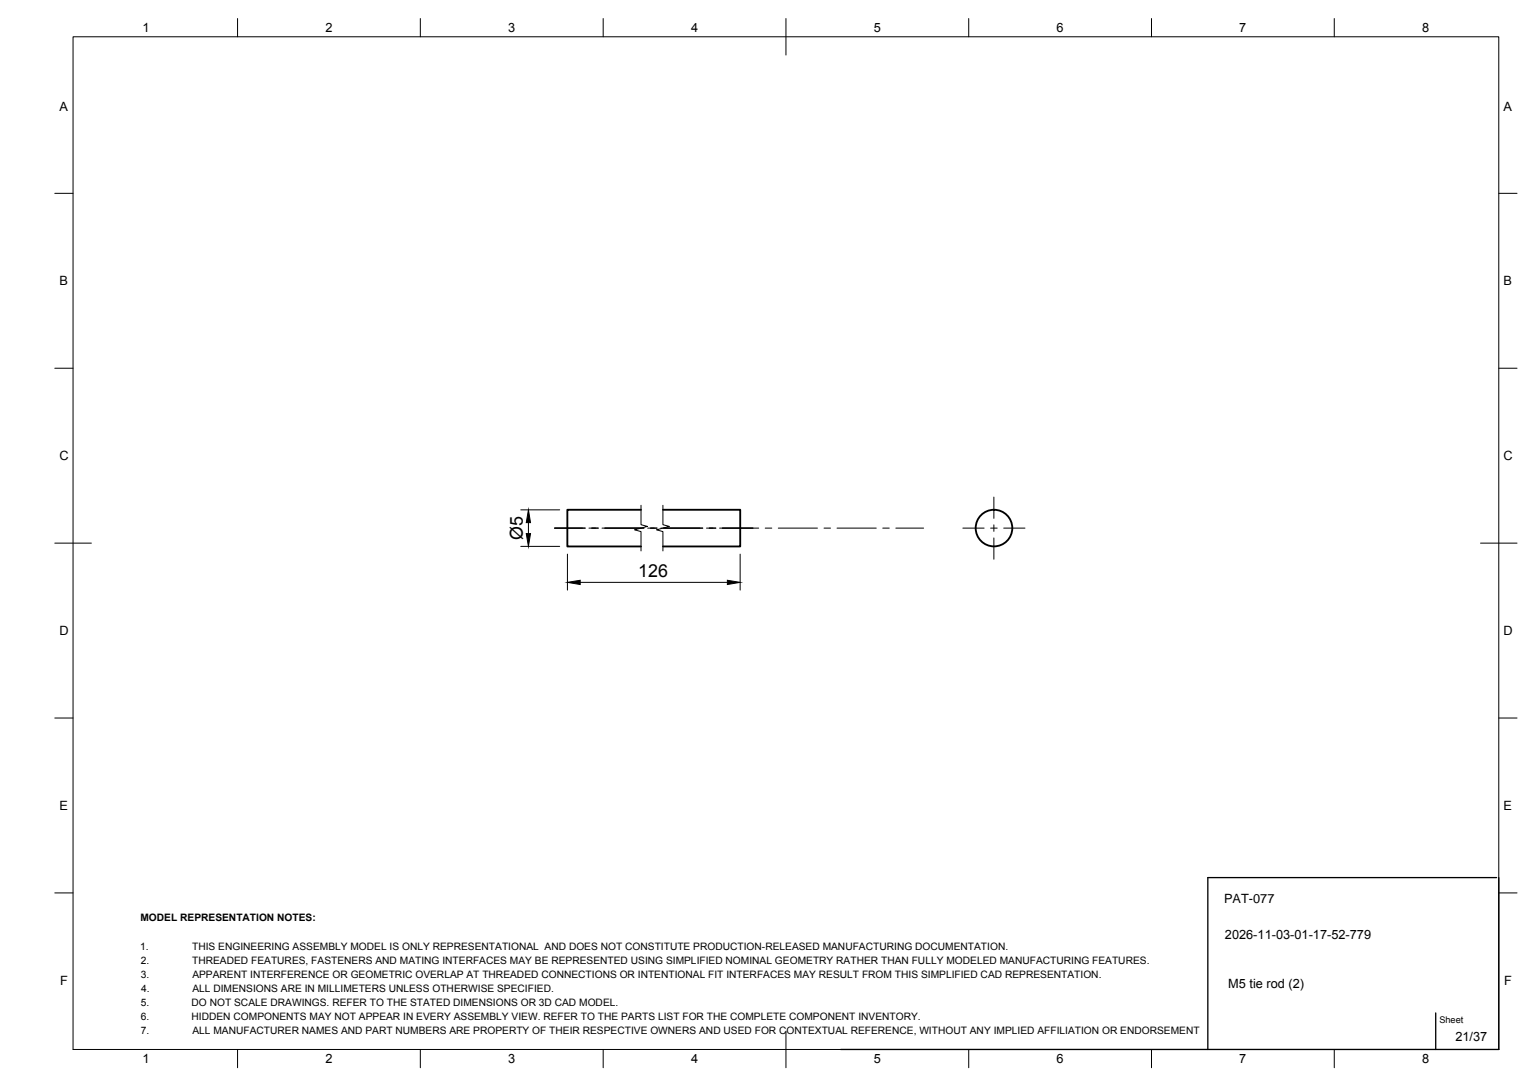
ISO-10303-21;
HEADER;
/* Generated by software containing ST-Developer
 * from STEP Tools, Inc. (www.steptools.com) 
 */

FILE_DESCRIPTION(
/* description */ ('Pallet stop with pneumatic fitting'),
/* implementation_level */ '2;1');

FILE_NAME(
/* name */ 'M5 tie rod (2).step',
/* time_stamp */ '2026-10-27T10:51:41-07:00',
/* author */ (''),
/* organization */ (''),
/* preprocessor_version */ 'ST-DEVELOPER v20.2',
/* originating_system */ 'Autodesk Translation Framework v15.17.0.0',
/* authorisation */ '');

FILE_SCHEMA (('AUTOMOTIVE_DESIGN { 1 0 10303 214 3 1 1 }'));
ENDSEC;

DATA;
#10=MECHANICAL_DESIGN_GEOMETRIC_PRESENTATION_REPRESENTATION('',(#373),#10265);
#309=SHAPE_REPRESENTATION_RELATIONSHIP('SRR','None',#10422,#341);
#341=ADVANCED_BREP_SHAPE_REPRESENTATION('',(#405),#10246);
#373=STYLED_ITEM('',(#10655),#405);
#405=MANIFOLD_SOLID_BREP('Body1',#5061);
#628=PLANE('',#5743);
#629=PLANE('',#5744);
#888=FACE_OUTER_BOUND('',#1287,.T.);
#889=FACE_OUTER_BOUND('',#1288,.T.);
#890=FACE_OUTER_BOUND('',#1289,.T.);
#1287=EDGE_LOOP('',(#3988,#3989,#3990,#3991));
#1288=EDGE_LOOP('',(#3992));
#1289=EDGE_LOOP('',(#3993));
#1634=LINE('',#9346,#1969);
#1969=VECTOR('',#6853,0.25);
#2298=CIRCLE('',#5741,0.25);
#2299=CIRCLE('',#5742,0.25);
#2598=VERTEX_POINT('',#9343);
#2599=VERTEX_POINT('',#9345);
#3093=EDGE_CURVE('',#2598,#2598,#2298,.T.);
#3094=EDGE_CURVE('',#2598,#2599,#1634,.T.);
#3095=EDGE_CURVE('',#2599,#2599,#2299,.T.);
#3988=ORIENTED_EDGE('',*,*,#3093,.F.);
#3989=ORIENTED_EDGE('',*,*,#3094,.T.);
#3990=ORIENTED_EDGE('',*,*,#3095,.T.);
#3991=ORIENTED_EDGE('',*,*,#3094,.F.);
#3992=ORIENTED_EDGE('',*,*,#3093,.T.);
#3993=ORIENTED_EDGE('',*,*,#3095,.F.);
#4690=CYLINDRICAL_SURFACE('',#5740,0.25);
#4883=ADVANCED_FACE('',(#888),#4690,.T.);
#4884=ADVANCED_FACE('',(#889),#628,.T.);
#4885=ADVANCED_FACE('',(#890),#629,.F.);
#5061=CLOSED_SHELL('',(#4883,#4884,#4885));
#5739=AXIS2_PLACEMENT_3D('',#9341,#6847,#6848);
#5740=AXIS2_PLACEMENT_3D('',#9342,#6849,#6850);
#5741=AXIS2_PLACEMENT_3D('',#9344,#6851,#6852);
#5742=AXIS2_PLACEMENT_3D('',#9347,#6854,#6855);
#5743=AXIS2_PLACEMENT_3D('',#9348,#6856,#6857);
#5744=AXIS2_PLACEMENT_3D('',#9349,#6858,#6859);
#6847=DIRECTION('axis',(0.,0.,1.));
#6848=DIRECTION('refdir',(1.,0.,0.));
#6849=DIRECTION('center_axis',(0.,0.,1.));
#6850=DIRECTION('ref_axis',(1.,0.,0.));
#6851=DIRECTION('center_axis',(0.,0.,1.));
#6852=DIRECTION('ref_axis',(1.,0.,0.));
#6853=DIRECTION('',(0.,0.,-1.));
#6854=DIRECTION('center_axis',(0.,0.,1.));
#6855=DIRECTION('ref_axis',(1.,0.,0.));
#6856=DIRECTION('center_axis',(0.,0.,1.));
#6857=DIRECTION('ref_axis',(1.,0.,0.));
#6858=DIRECTION('center_axis',(0.,0.,1.));
#6859=DIRECTION('ref_axis',(1.,0.,0.));
#9341=CARTESIAN_POINT('',(0.,0.,0.));
#9342=CARTESIAN_POINT('Origin',(2.72720779386421,2.72720779386421,-1.8));
#9343=CARTESIAN_POINT('',(2.47720779386421,2.72720779386421,10.8));
#9344=CARTESIAN_POINT('Origin',(2.72720779386421,2.72720779386421,10.8));
#9345=CARTESIAN_POINT('',(2.47720779386421,2.72720779386421,-1.8));
#9346=CARTESIAN_POINT('',(2.47720779386421,2.72720779386421,-1.8));
#9347=CARTESIAN_POINT('Origin',(2.72720779386421,2.72720779386421,-1.8));
#9348=CARTESIAN_POINT('Origin',(2.72720779386421,2.72720779386421,10.8));
#9349=CARTESIAN_POINT('Origin',(2.72720779386421,2.72720779386421,-1.8));
#10208=UNCERTAINTY_MEASURE_WITH_UNIT(LENGTH_MEASURE(0.001),#10266,
'DISTANCE_ACCURACY_VALUE',
'Maximum model space distance between geometric entities at asserted c
onnectivities');
#10227=UNCERTAINTY_MEASURE_WITH_UNIT(LENGTH_MEASURE(0.001),#10266,
'DISTANCE_ACCURACY_VALUE',
'Maximum model space distance between geometric entities at asserted c
onnectivities');
#10246=(
GEOMETRIC_REPRESENTATION_CONTEXT(3)
GLOBAL_UNCERTAINTY_ASSIGNED_CONTEXT((#10208))
GLOBAL_UNIT_ASSIGNED_CONTEXT((#10266,#10268,#10269))
REPRESENTATION_CONTEXT('','3D')
);
#10265=(
GEOMETRIC_REPRESENTATION_CONTEXT(3)
GLOBAL_UNCERTAINTY_ASSIGNED_CONTEXT((#10227))
GLOBAL_UNIT_ASSIGNED_CONTEXT((#10266,#10268,#10269))
REPRESENTATION_CONTEXT('','3D')
);
#10266=(
LENGTH_UNIT()
NAMED_UNIT(*)
SI_UNIT(.CENTI.,.METRE.)
);
#10268=(
NAMED_UNIT(*)
PLANE_ANGLE_UNIT()
SI_UNIT($,.RADIAN.)
);
#10269=(
NAMED_UNIT(*)
SI_UNIT($,.STERADIAN.)
SOLID_ANGLE_UNIT()
);
#10288=SHAPE_DEFINITION_REPRESENTATION(#10325,#10422);
#10325=PRODUCT_DEFINITION_SHAPE('',$,#10460);
#10422=SHAPE_REPRESENTATION('',(#5739),#10246);
#10441=PRODUCT_DEFINITION_CONTEXT('part definition',#10554,'design');
#10460=PRODUCT_DEFINITION('M5 tie rod (2)','M5 tie rod (2)',#10497,#10441);
#10497=PRODUCT_DEFINITION_FORMATION('',$,#10574);
#10554=APPLICATION_CONTEXT(
'Core Data for Automotive Mechanical Design Process');
#10555=PRODUCT_CONTEXT('part definition',#10554,'mechanical');
#10574=PRODUCT('M5 tie rod (2)','M5 tie rod (2)','M5 tie rod (2)',(#10555));
#10649=COLOUR_RGB('Grey',0.48,0.52,0.57);
#10650=FILL_AREA_STYLE_COLOUR('',#10649);
#10651=FILL_AREA_STYLE('',(#10650));
#10652=SURFACE_STYLE_FILL_AREA(#10651);
#10653=SURFACE_SIDE_STYLE('',(#10652));
#10654=SURFACE_STYLE_USAGE(.BOTH.,#10653);
#10655=PRESENTATION_STYLE_ASSIGNMENT((#10654));
ENDSEC;
END-ISO-10303-21;
